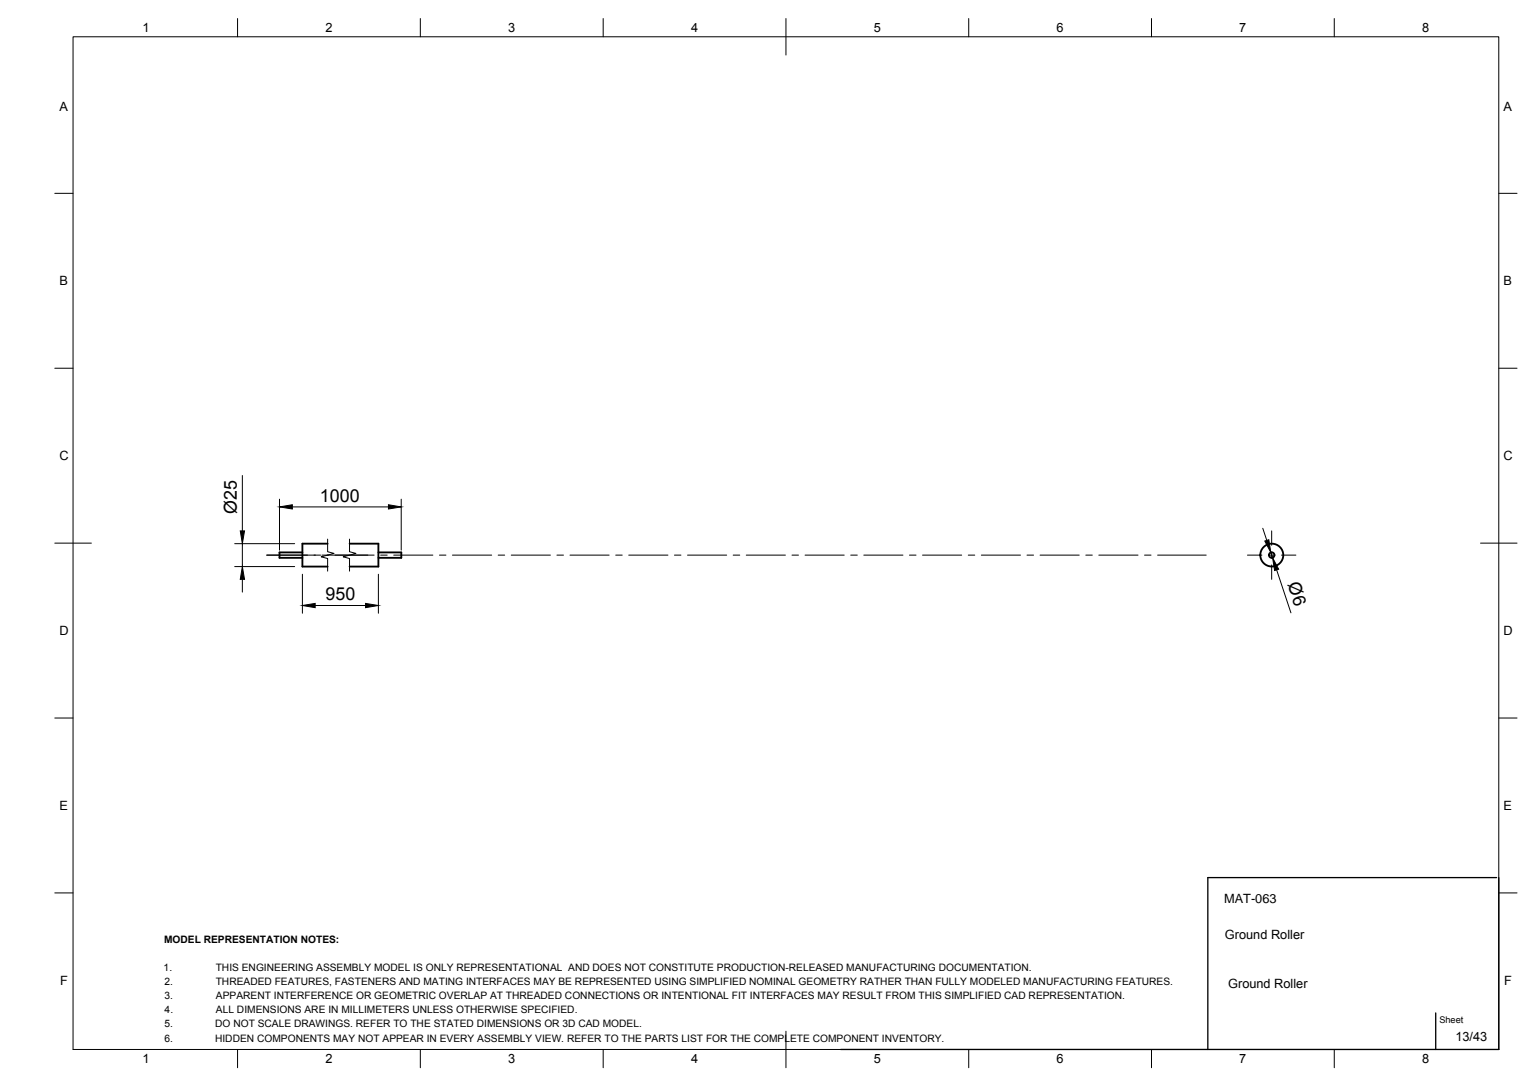
ISO-10303-21;
HEADER;
/* Generated by software containing ST-Developer
 * from STEP Tools, Inc. (www.steptools.com) 
 */

FILE_DESCRIPTION(
/* description */ (''),
/* implementation_level */ '2;1');

FILE_NAME(
/* name */ 'Ground Roller.step',
/* time_stamp */ '2026-10-24T09:43:01-07:00',
/* author */ (''),
/* organization */ (''),
/* preprocessor_version */ 'ST-DEVELOPER v20.2',
/* originating_system */ 'Autodesk Translation Framework v15.15.0.0',
/* authorisation */ '');

FILE_SCHEMA (('AUTOMOTIVE_DESIGN { 1 0 10303 214 3 1 1 }'));
ENDSEC;

DATA;
#10=MECHANICAL_DESIGN_GEOMETRIC_PRESENTATION_REPRESENTATION('',(#290),#11112);
#224=SHAPE_REPRESENTATION_RELATIONSHIP('SRR','None',#11248,#257);
#257=ADVANCED_BREP_SHAPE_REPRESENTATION('',(#323),#11093);
#290=STYLED_ITEM('',(#11426),#323);
#323=MANIFOLD_SOLID_BREP('Ground Roller',#6027);
#453=FACE_BOUND('',#1417,.T.);
#454=FACE_BOUND('',#1420,.T.);
#606=PLANE('',#7034);
#607=PLANE('',#7035);
#608=PLANE('',#7039);
#609=PLANE('',#7043);
#936=FACE_OUTER_BOUND('',#1414,.T.);
#937=FACE_OUTER_BOUND('',#1415,.T.);
#938=FACE_OUTER_BOUND('',#1416,.T.);
#939=FACE_OUTER_BOUND('',#1418,.T.);
#940=FACE_OUTER_BOUND('',#1419,.T.);
#941=FACE_OUTER_BOUND('',#1421,.T.);
#942=FACE_OUTER_BOUND('',#1422,.T.);
#1414=EDGE_LOOP('',(#5095,#5096,#5097,#5098));
#1415=EDGE_LOOP('',(#5099));
#1416=EDGE_LOOP('',(#5100));
#1417=EDGE_LOOP('',(#5101));
#1418=EDGE_LOOP('',(#5102,#5103,#5104,#5105));
#1419=EDGE_LOOP('',(#5106));
#1420=EDGE_LOOP('',(#5107));
#1421=EDGE_LOOP('',(#5108,#5109,#5110,#5111));
#1422=EDGE_LOOP('',(#5112));
#1795=LINE('',#10552,#2154);
#1796=LINE('',#10561,#2155);
#1797=LINE('',#10568,#2156);
#2154=VECTOR('',#8749,0.003);
#2155=VECTOR('',#8762,0.0125);
#2156=VECTOR('',#8771,0.003);
#2610=CIRCLE('',#7032,0.003);
#2611=CIRCLE('',#7033,0.003);
#2612=CIRCLE('',#7036,0.0125);
#2613=CIRCLE('',#7038,0.0125);
#2614=CIRCLE('',#7040,0.003);
#2615=CIRCLE('',#7042,0.003);
#3044=VERTEX_POINT('',#10549);
#3045=VERTEX_POINT('',#10551);
#3046=VERTEX_POINT('',#10556);
#3047=VERTEX_POINT('',#10559);
#3048=VERTEX_POINT('',#10563);
#3049=VERTEX_POINT('',#10566);
#3751=EDGE_CURVE('',#3044,#3044,#2610,.F.);
#3752=EDGE_CURVE('',#3044,#3045,#1795,.T.);
#3753=EDGE_CURVE('',#3045,#3045,#2611,.T.);
#3754=EDGE_CURVE('',#3046,#3046,#2612,.F.);
#3755=EDGE_CURVE('',#3047,#3047,#2613,.F.);
#3756=EDGE_CURVE('',#3047,#3046,#1796,.T.);
#3757=EDGE_CURVE('',#3048,#3048,#2614,.T.);
#3758=EDGE_CURVE('',#3049,#3049,#2615,.F.);
#3759=EDGE_CURVE('',#3049,#3048,#1797,.T.);
#5095=ORIENTED_EDGE('',*,*,#3751,.T.);
#5096=ORIENTED_EDGE('',*,*,#3752,.T.);
#5097=ORIENTED_EDGE('',*,*,#3753,.T.);
#5098=ORIENTED_EDGE('',*,*,#3752,.F.);
#5099=ORIENTED_EDGE('',*,*,#3753,.F.);
#5100=ORIENTED_EDGE('',*,*,#3754,.T.);
#5101=ORIENTED_EDGE('',*,*,#3751,.F.);
#5102=ORIENTED_EDGE('',*,*,#3755,.T.);
#5103=ORIENTED_EDGE('',*,*,#3756,.T.);
#5104=ORIENTED_EDGE('',*,*,#3754,.F.);
#5105=ORIENTED_EDGE('',*,*,#3756,.F.);
#5106=ORIENTED_EDGE('',*,*,#3755,.F.);
#5107=ORIENTED_EDGE('',*,*,#3757,.F.);
#5108=ORIENTED_EDGE('',*,*,#3758,.T.);
#5109=ORIENTED_EDGE('',*,*,#3759,.T.);
#5110=ORIENTED_EDGE('',*,*,#3757,.T.);
#5111=ORIENTED_EDGE('',*,*,#3759,.F.);
#5112=ORIENTED_EDGE('',*,*,#3758,.F.);
#5604=CYLINDRICAL_SURFACE('',#7031,0.003);
#5605=CYLINDRICAL_SURFACE('',#7037,0.0125);
#5606=CYLINDRICAL_SURFACE('',#7041,0.003);
#5909=ADVANCED_FACE('',(#936),#5604,.T.);
#5910=ADVANCED_FACE('',(#937),#606,.T.);
#5911=ADVANCED_FACE('',(#938,#453),#607,.T.);
#5912=ADVANCED_FACE('',(#939),#5605,.T.);
#5913=ADVANCED_FACE('',(#940,#454),#608,.F.);
#5914=ADVANCED_FACE('',(#941),#5606,.T.);
#5915=ADVANCED_FACE('',(#942),#609,.F.);
#6027=CLOSED_SHELL('',(#5909,#5910,#5911,#5912,#5913,#5914,#5915));
#7030=AXIS2_PLACEMENT_3D('',#10547,#8743,#8744);
#7031=AXIS2_PLACEMENT_3D('',#10548,#8745,#8746);
#7032=AXIS2_PLACEMENT_3D('',#10550,#8747,#8748);
#7033=AXIS2_PLACEMENT_3D('',#10553,#8750,#8751);
#7034=AXIS2_PLACEMENT_3D('',#10554,#8752,#8753);
#7035=AXIS2_PLACEMENT_3D('',#10555,#8754,#8755);
#7036=AXIS2_PLACEMENT_3D('',#10557,#8756,#8757);
#7037=AXIS2_PLACEMENT_3D('',#10558,#8758,#8759);
#7038=AXIS2_PLACEMENT_3D('',#10560,#8760,#8761);
#7039=AXIS2_PLACEMENT_3D('',#10562,#8763,#8764);
#7040=AXIS2_PLACEMENT_3D('',#10564,#8765,#8766);
#7041=AXIS2_PLACEMENT_3D('',#10565,#8767,#8768);
#7042=AXIS2_PLACEMENT_3D('',#10567,#8769,#8770);
#7043=AXIS2_PLACEMENT_3D('',#10569,#8772,#8773);
#8743=DIRECTION('axis',(0.,0.,1.));
#8744=DIRECTION('refdir',(1.,0.,0.));
#8745=DIRECTION('center_axis',(-1.,0.,0.));
#8746=DIRECTION('ref_axis',(0.,0.,1.));
#8747=DIRECTION('center_axis',(-1.,0.,0.));
#8748=DIRECTION('ref_axis',(0.,0.,1.));
#8749=DIRECTION('',(1.,0.,0.));
#8750=DIRECTION('center_axis',(-1.,0.,0.));
#8751=DIRECTION('ref_axis',(0.,0.,1.));
#8752=DIRECTION('center_axis',(1.,0.,0.));
#8753=DIRECTION('ref_axis',(0.,0.,-1.));
#8754=DIRECTION('center_axis',(1.,2.02536400451272E-15,-2.2981616621275E-15));
#8755=DIRECTION('ref_axis',(-2.2981616621275E-15,0.,-1.));
#8756=DIRECTION('center_axis',(-1.,0.,0.));
#8757=DIRECTION('ref_axis',(0.,0.,1.));
#8758=DIRECTION('center_axis',(-1.,0.,0.));
#8759=DIRECTION('ref_axis',(0.,0.,1.));
#8760=DIRECTION('center_axis',(-1.,0.,0.));
#8761=DIRECTION('ref_axis',(0.,0.,1.));
#8762=DIRECTION('',(1.,0.,0.));
#8763=DIRECTION('center_axis',(1.,-2.02536400451272E-15,2.2981616621275E-15));
#8764=DIRECTION('ref_axis',(2.2981616621275E-15,0.,-1.));
#8765=DIRECTION('center_axis',(-1.,0.,0.));
#8766=DIRECTION('ref_axis',(0.,0.,1.));
#8767=DIRECTION('center_axis',(-1.,0.,0.));
#8768=DIRECTION('ref_axis',(0.,0.,1.));
#8769=DIRECTION('center_axis',(-1.,0.,0.));
#8770=DIRECTION('ref_axis',(0.,0.,1.));
#8771=DIRECTION('',(1.,0.,0.));
#8772=DIRECTION('center_axis',(1.,0.,0.));
#8773=DIRECTION('ref_axis',(0.,0.,-1.));
#10547=CARTESIAN_POINT('',(0.,0.,0.));
#10548=CARTESIAN_POINT('Origin',(0.5,-0.549047301,0.966510346));
#10549=CARTESIAN_POINT('',(0.475,-0.549047301,0.963510346));
#10550=CARTESIAN_POINT('Origin',(0.475,-0.549047301,0.966510346));
#10551=CARTESIAN_POINT('',(0.5,-0.549047301,0.963510346));
#10552=CARTESIAN_POINT('',(0.5,-0.549047301,0.963510346));
#10553=CARTESIAN_POINT('Origin',(0.5,-0.549047301,0.966510346));
#10554=CARTESIAN_POINT('Origin',(0.5,-0.549047301000001,0.966510346));
#10555=CARTESIAN_POINT('Origin',(0.475,-0.549047301,0.966510346));
#10556=CARTESIAN_POINT('',(0.475,-0.549047301,0.954010346));
#10557=CARTESIAN_POINT('Origin',(0.475,-0.549047301,0.966510346));
#10558=CARTESIAN_POINT('Origin',(0.475,-0.549047301,0.966510346));
#10559=CARTESIAN_POINT('',(-0.475,-0.549047301,0.954010346));
#10560=CARTESIAN_POINT('Origin',(-0.475,-0.549047301,0.966510346));
#10561=CARTESIAN_POINT('',(0.475,-0.549047301,0.954010346));
#10562=CARTESIAN_POINT('Origin',(-0.475,-0.549047301,0.966510346));
#10563=CARTESIAN_POINT('',(-0.475,-0.549047301,0.963510346));
#10564=CARTESIAN_POINT('Origin',(-0.475,-0.549047301,0.966510346));
#10565=CARTESIAN_POINT('Origin',(0.5,-0.549047301,0.966510346));
#10566=CARTESIAN_POINT('',(-0.5,-0.549047301,0.963510346));
#10567=CARTESIAN_POINT('Origin',(-0.5,-0.549047301,0.966510346));
#10568=CARTESIAN_POINT('',(0.5,-0.549047301,0.963510346));
#10569=CARTESIAN_POINT('Origin',(-0.5,-0.549047301000001,0.966510346));
#11054=UNCERTAINTY_MEASURE_WITH_UNIT(LENGTH_MEASURE(1.E-5),#11113,
'DISTANCE_ACCURACY_VALUE',
'Maximum model space distance between geometric entities at asserted c
onnectivities');
#11073=UNCERTAINTY_MEASURE_WITH_UNIT(LENGTH_MEASURE(1.E-5),#11113,
'DISTANCE_ACCURACY_VALUE',
'Maximum model space distance between geometric entities at asserted c
onnectivities');
#11093=(
GEOMETRIC_REPRESENTATION_CONTEXT(3)
GLOBAL_UNCERTAINTY_ASSIGNED_CONTEXT((#11054))
GLOBAL_UNIT_ASSIGNED_CONTEXT((#11113,#11114,#11115))
REPRESENTATION_CONTEXT('','3D')
);
#11112=(
GEOMETRIC_REPRESENTATION_CONTEXT(3)
GLOBAL_UNCERTAINTY_ASSIGNED_CONTEXT((#11073))
GLOBAL_UNIT_ASSIGNED_CONTEXT((#11113,#11114,#11115))
REPRESENTATION_CONTEXT('','3D')
);
#11113=(
LENGTH_UNIT()
NAMED_UNIT(*)
SI_UNIT($,.METRE.)
);
#11114=(
NAMED_UNIT(*)
PLANE_ANGLE_UNIT()
SI_UNIT($,.RADIAN.)
);
#11115=(
NAMED_UNIT(*)
SI_UNIT($,.STERADIAN.)
SOLID_ANGLE_UNIT()
);
#11135=SHAPE_DEFINITION_REPRESENTATION(#11180,#11248);
#11180=PRODUCT_DEFINITION_SHAPE('',$,#11287);
#11248=SHAPE_REPRESENTATION('',(#7030),#11093);
#11267=PRODUCT_DEFINITION_CONTEXT('part definition',#11383,'design');
#11287=PRODUCT_DEFINITION('Ground Roller','Ground Roller',#11325,#11267);
#11325=PRODUCT_DEFINITION_FORMATION('',$,#11404);
#11383=APPLICATION_CONTEXT(
'Core Data for Automotive Mechanical Design Process');
#11384=PRODUCT_CONTEXT('part definition',#11383,'mechanical');
#11404=PRODUCT('Ground Roller','Ground Roller',
'ground_roller__ DE     8465',(#11384));
#11426=PRESENTATION_STYLE_ASSIGNMENT((#11430));
#11430=SURFACE_STYLE_USAGE(.BOTH.,#11434);
#11434=SURFACE_SIDE_STYLE('',(#11438));
#11438=SURFACE_STYLE_FILL_AREA(#11442);
#11442=FILL_AREA_STYLE('Opaque(202,209,238)',(#11446));
#11446=FILL_AREA_STYLE_COLOUR('Opaque(202,209,238)',#11450);
#11450=COLOUR_RGB('Opaque(202,209,238)',0.792156862745098,0.819607843137255,
0.933333333333333);
ENDSEC;
END-ISO-10303-21;
